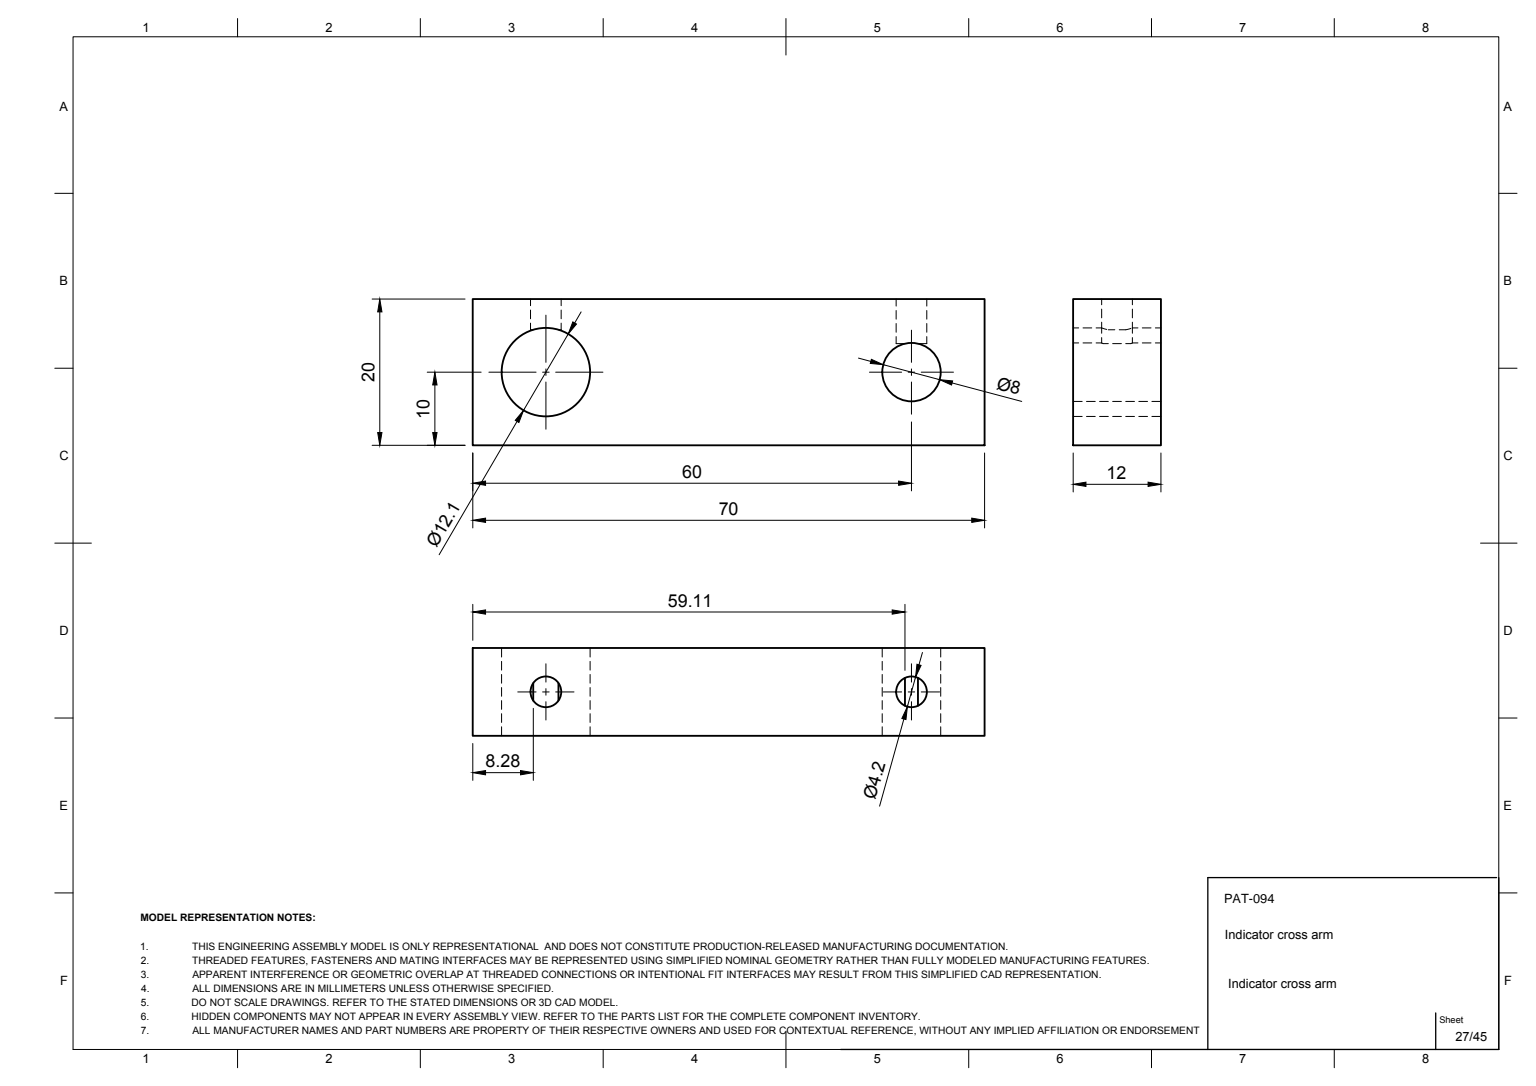
ISO-10303-21;
HEADER;
/* Generated by software containing ST-Developer
 * from STEP Tools, Inc. (www.steptools.com) 
 */

FILE_DESCRIPTION(
/* description */ ('Shaft runout checking stand'),
/* implementation_level */ '2;1');

FILE_NAME(
/* name */ 'Indicator cross arm.step',
/* time_stamp */ '2026-11-02T21:12:33-08:00',
/* author */ (''),
/* organization */ (''),
/* preprocessor_version */ 'ST-DEVELOPER v20.2',
/* originating_system */ 'Autodesk Translation Framework v15.17.0.0',
/* authorisation */ '');

FILE_SCHEMA (('AUTOMOTIVE_DESIGN { 1 0 10303 214 3 1 1 }'));
ENDSEC;

DATA;
#10=MECHANICAL_DESIGN_GEOMETRIC_PRESENTATION_REPRESENTATION('',(#488),#11748);
#329=B_SPLINE_CURVE_WITH_KNOTS('',3,(#10633,#10634,#10635,#10636,#10637,
#10638,#10639,#10640,#10641,#10642),.UNSPECIFIED.,.F.,.F.,(4,2,2,2,4),(0.882019934661292,
0.890219855506043,0.970998038219416,1.05177622093279,1.05997614177754),
 .UNSPECIFIED.);
#330=B_SPLINE_CURVE_WITH_KNOTS('',3,(#10645,#10646,#10647,#10648,#10649,
#10650,#10651,#10652,#10653,#10654),.UNSPECIFIED.,.F.,.F.,(4,2,2,2,4),(0.234687909181681,
0.242887830026432,0.323666012739805,0.404444195453179,0.41264411629793),
 .UNSPECIFIED.);
#331=B_SPLINE_CURVE_WITH_KNOTS('',3,(#10669,#10670,#10671,#10672,#10673,
#10674,#10675,#10676,#10677,#10678,#10679,#10680,#10681,#10682),
 .UNSPECIFIED.,.F.,.F.,(4,2,2,2,2,2,4),(0.761877411255191,0.798325568640294,
0.878131747417165,0.957937926194035,1.03774410497091,1.11755028374778,1.15399844113288),
 .UNSPECIFIED.);
#332=B_SPLINE_CURVE_WITH_KNOTS('',3,(#10685,#10686,#10687,#10688,#10689,
#10690,#10691,#10692,#10693,#10694,#10695,#10696,#10697,#10698),
 .UNSPECIFIED.,.F.,.F.,(4,2,2,2,2,2,4),(0.123252127125832,0.159700284510937,
0.239506463287808,0.319312642064678,0.399118820841549,0.47892499961842,
0.515373157003523),.UNSPECIFIED.);
#402=SHAPE_REPRESENTATION_RELATIONSHIP('SRR','None',#11951,#445);
#445=ADVANCED_BREP_SHAPE_REPRESENTATION('',(#536),#11727);
#488=STYLED_ITEM('',(#12169),#536);
#536=MANIFOLD_SOLID_BREP('Body1',#6234);
#641=FACE_BOUND('',#1738,.T.);
#642=FACE_BOUND('',#1740,.T.);
#643=FACE_BOUND('',#1742,.T.);
#644=FACE_BOUND('',#1743,.T.);
#645=FACE_BOUND('',#1748,.T.);
#646=FACE_BOUND('',#1749,.T.);
#647=FACE_BOUND('',#1751,.T.);
#648=FACE_BOUND('',#1752,.T.);
#815=CIRCLE('',#7153,0.21);
#816=CIRCLE('',#7154,0.21);
#817=CIRCLE('',#7156,0.21);
#818=CIRCLE('',#7157,0.21);
#819=CIRCLE('',#7160,0.21);
#820=CIRCLE('',#7161,0.21);
#821=CIRCLE('',#7163,0.21);
#822=CIRCLE('',#7164,0.21);
#823=CIRCLE('',#7167,0.4);
#824=CIRCLE('',#7168,0.4);
#825=CIRCLE('',#7170,0.605);
#826=CIRCLE('',#7171,0.605);
#1003=CYLINDRICAL_SURFACE('',#7155,0.21);
#1004=CYLINDRICAL_SURFACE('',#7162,0.21);
#1005=CYLINDRICAL_SURFACE('',#7166,0.4);
#1006=CYLINDRICAL_SURFACE('',#7169,0.605);
#1284=FACE_OUTER_BOUND('',#1731,.T.);
#1285=FACE_OUTER_BOUND('',#1732,.T.);
#1286=FACE_OUTER_BOUND('',#1733,.T.);
#1287=FACE_OUTER_BOUND('',#1734,.T.);
#1288=FACE_OUTER_BOUND('',#1735,.T.);
#1289=FACE_OUTER_BOUND('',#1736,.T.);
#1290=FACE_OUTER_BOUND('',#1737,.T.);
#1291=FACE_OUTER_BOUND('',#1739,.T.);
#1292=FACE_OUTER_BOUND('',#1741,.T.);
#1293=FACE_OUTER_BOUND('',#1744,.T.);
#1294=FACE_OUTER_BOUND('',#1745,.T.);
#1295=FACE_OUTER_BOUND('',#1746,.T.);
#1296=FACE_OUTER_BOUND('',#1747,.T.);
#1297=FACE_OUTER_BOUND('',#1750,.T.);
#1731=EDGE_LOOP('',(#5142,#5143,#5144));
#1732=EDGE_LOOP('',(#5145,#5146,#5147,#5148,#5149,#5150,#5151,#5152));
#1733=EDGE_LOOP('',(#5153,#5154));
#1734=EDGE_LOOP('',(#5155,#5156,#5157));
#1735=EDGE_LOOP('',(#5158,#5159,#5160,#5161,#5162,#5163,#5164,#5165));
#1736=EDGE_LOOP('',(#5166,#5167));
#1737=EDGE_LOOP('',(#5168,#5169,#5170,#5171));
#1738=EDGE_LOOP('',(#5172,#5173,#5174,#5175));
#1739=EDGE_LOOP('',(#5176,#5177,#5178,#5179));
#1740=EDGE_LOOP('',(#5180,#5181,#5182,#5183));
#1741=EDGE_LOOP('',(#5184,#5185,#5186,#5187));
#1742=EDGE_LOOP('',(#5188));
#1743=EDGE_LOOP('',(#5189));
#1744=EDGE_LOOP('',(#5190,#5191,#5192,#5193));
#1745=EDGE_LOOP('',(#5194,#5195,#5196,#5197));
#1746=EDGE_LOOP('',(#5198,#5199,#5200,#5201));
#1747=EDGE_LOOP('',(#5202,#5203,#5204,#5205));
#1748=EDGE_LOOP('',(#5206));
#1749=EDGE_LOOP('',(#5207));
#1750=EDGE_LOOP('',(#5208,#5209,#5210,#5211));
#1751=EDGE_LOOP('',(#5212));
#1752=EDGE_LOOP('',(#5213));
#2268=LINE('',#10627,#2735);
#2269=LINE('',#10656,#2736);
#2270=LINE('',#10659,#2737);
#2271=LINE('',#10663,#2738);
#2272=LINE('',#10700,#2739);
#2273=LINE('',#10703,#2740);
#2274=LINE('',#10708,#2741);
#2275=LINE('',#10714,#2742);
#2276=LINE('',#10719,#2743);
#2277=LINE('',#10721,#2744);
#2278=LINE('',#10723,#2745);
#2279=LINE('',#10724,#2746);
#2280=LINE('',#10727,#2747);
#2281=LINE('',#10729,#2748);
#2282=LINE('',#10730,#2749);
#2283=LINE('',#10733,#2750);
#2284=LINE('',#10735,#2751);
#2285=LINE('',#10736,#2752);
#2286=LINE('',#10738,#2753);
#2287=LINE('',#10739,#2754);
#2735=VECTOR('',#8713,1.);
#2736=VECTOR('',#8722,0.21);
#2737=VECTOR('',#8727,1.);
#2738=VECTOR('',#8730,1.);
#2739=VECTOR('',#8739,0.21);
#2740=VECTOR('',#8744,1.);
#2741=VECTOR('',#8749,0.4);
#2742=VECTOR('',#8756,0.605000000000001);
#2743=VECTOR('',#8761,1.);
#2744=VECTOR('',#8762,1.);
#2745=VECTOR('',#8763,1.);
#2746=VECTOR('',#8764,1.);
#2747=VECTOR('',#8767,1.);
#2748=VECTOR('',#8768,1.);
#2749=VECTOR('',#8769,1.);
#2750=VECTOR('',#8772,1.);
#2751=VECTOR('',#8773,1.);
#2752=VECTOR('',#8774,1.);
#2753=VECTOR('',#8777,1.);
#2754=VECTOR('',#8778,1.);
#3167=VERTEX_POINT('',#10625);
#3168=VERTEX_POINT('',#10626);
#3169=VERTEX_POINT('',#10628);
#3170=VERTEX_POINT('',#10632);
#3171=VERTEX_POINT('',#10643);
#3172=VERTEX_POINT('',#10655);
#3173=VERTEX_POINT('',#10661);
#3174=VERTEX_POINT('',#10662);
#3175=VERTEX_POINT('',#10664);
#3176=VERTEX_POINT('',#10668);
#3177=VERTEX_POINT('',#10683);
#3178=VERTEX_POINT('',#10699);
#3179=VERTEX_POINT('',#10705);
#3180=VERTEX_POINT('',#10707);
#3181=VERTEX_POINT('',#10711);
#3182=VERTEX_POINT('',#10713);
#3183=VERTEX_POINT('',#10717);
#3184=VERTEX_POINT('',#10718);
#3185=VERTEX_POINT('',#10720);
#3186=VERTEX_POINT('',#10722);
#3187=VERTEX_POINT('',#10726);
#3188=VERTEX_POINT('',#10728);
#3189=VERTEX_POINT('',#10732);
#3190=VERTEX_POINT('',#10734);
#3857=EDGE_CURVE('',#3167,#3168,#2268,.T.);
#3858=EDGE_CURVE('',#3167,#3169,#815,.T.);
#3859=EDGE_CURVE('',#3169,#3168,#816,.T.);
#3860=EDGE_CURVE('',#3170,#3167,#329,.T.);
#3861=EDGE_CURVE('',#3171,#3170,#817,.T.);
#3862=EDGE_CURVE('',#3168,#3171,#330,.T.);
#3863=EDGE_CURVE('',#3169,#3172,#2269,.T.);
#3864=EDGE_CURVE('',#3172,#3172,#818,.T.);
#3865=EDGE_CURVE('',#3171,#3170,#2270,.T.);
#3866=EDGE_CURVE('',#3173,#3174,#2271,.T.);
#3867=EDGE_CURVE('',#3173,#3175,#819,.T.);
#3868=EDGE_CURVE('',#3175,#3174,#820,.T.);
#3869=EDGE_CURVE('',#3176,#3173,#331,.T.);
#3870=EDGE_CURVE('',#3177,#3176,#821,.T.);
#3871=EDGE_CURVE('',#3174,#3177,#332,.T.);
#3872=EDGE_CURVE('',#3175,#3178,#2272,.T.);
#3873=EDGE_CURVE('',#3178,#3178,#822,.T.);
#3874=EDGE_CURVE('',#3177,#3176,#2273,.T.);
#3875=EDGE_CURVE('',#3179,#3179,#823,.T.);
#3876=EDGE_CURVE('',#3179,#3180,#2274,.T.);
#3877=EDGE_CURVE('',#3180,#3180,#824,.T.);
#3878=EDGE_CURVE('',#3181,#3181,#825,.T.);
#3879=EDGE_CURVE('',#3181,#3182,#2275,.T.);
#3880=EDGE_CURVE('',#3182,#3182,#826,.T.);
#3881=EDGE_CURVE('',#3183,#3184,#2276,.T.);
#3882=EDGE_CURVE('',#3184,#3185,#2277,.T.);
#3883=EDGE_CURVE('',#3186,#3185,#2278,.T.);
#3884=EDGE_CURVE('',#3183,#3186,#2279,.T.);
#3885=EDGE_CURVE('',#3187,#3183,#2280,.T.);
#3886=EDGE_CURVE('',#3188,#3186,#2281,.T.);
#3887=EDGE_CURVE('',#3187,#3188,#2282,.T.);
#3888=EDGE_CURVE('',#3189,#3187,#2283,.T.);
#3889=EDGE_CURVE('',#3190,#3188,#2284,.T.);
#3890=EDGE_CURVE('',#3189,#3190,#2285,.T.);
#3891=EDGE_CURVE('',#3184,#3189,#2286,.T.);
#3892=EDGE_CURVE('',#3185,#3190,#2287,.T.);
#5142=ORIENTED_EDGE('',*,*,#3857,.F.);
#5143=ORIENTED_EDGE('',*,*,#3858,.T.);
#5144=ORIENTED_EDGE('',*,*,#3859,.T.);
#5145=ORIENTED_EDGE('',*,*,#3860,.F.);
#5146=ORIENTED_EDGE('',*,*,#3861,.F.);
#5147=ORIENTED_EDGE('',*,*,#3862,.F.);
#5148=ORIENTED_EDGE('',*,*,#3859,.F.);
#5149=ORIENTED_EDGE('',*,*,#3863,.T.);
#5150=ORIENTED_EDGE('',*,*,#3864,.F.);
#5151=ORIENTED_EDGE('',*,*,#3863,.F.);
#5152=ORIENTED_EDGE('',*,*,#3858,.F.);
#5153=ORIENTED_EDGE('',*,*,#3865,.F.);
#5154=ORIENTED_EDGE('',*,*,#3861,.T.);
#5155=ORIENTED_EDGE('',*,*,#3866,.F.);
#5156=ORIENTED_EDGE('',*,*,#3867,.T.);
#5157=ORIENTED_EDGE('',*,*,#3868,.T.);
#5158=ORIENTED_EDGE('',*,*,#3869,.F.);
#5159=ORIENTED_EDGE('',*,*,#3870,.F.);
#5160=ORIENTED_EDGE('',*,*,#3871,.F.);
#5161=ORIENTED_EDGE('',*,*,#3868,.F.);
#5162=ORIENTED_EDGE('',*,*,#3872,.T.);
#5163=ORIENTED_EDGE('',*,*,#3873,.F.);
#5164=ORIENTED_EDGE('',*,*,#3872,.F.);
#5165=ORIENTED_EDGE('',*,*,#3867,.F.);
#5166=ORIENTED_EDGE('',*,*,#3874,.F.);
#5167=ORIENTED_EDGE('',*,*,#3870,.T.);
#5168=ORIENTED_EDGE('',*,*,#3875,.F.);
#5169=ORIENTED_EDGE('',*,*,#3876,.T.);
#5170=ORIENTED_EDGE('',*,*,#3877,.F.);
#5171=ORIENTED_EDGE('',*,*,#3876,.F.);
#5172=ORIENTED_EDGE('',*,*,#3862,.T.);
#5173=ORIENTED_EDGE('',*,*,#3865,.T.);
#5174=ORIENTED_EDGE('',*,*,#3860,.T.);
#5175=ORIENTED_EDGE('',*,*,#3857,.T.);
#5176=ORIENTED_EDGE('',*,*,#3878,.F.);
#5177=ORIENTED_EDGE('',*,*,#3879,.T.);
#5178=ORIENTED_EDGE('',*,*,#3880,.F.);
#5179=ORIENTED_EDGE('',*,*,#3879,.F.);
#5180=ORIENTED_EDGE('',*,*,#3871,.T.);
#5181=ORIENTED_EDGE('',*,*,#3874,.T.);
#5182=ORIENTED_EDGE('',*,*,#3869,.T.);
#5183=ORIENTED_EDGE('',*,*,#3866,.T.);
#5184=ORIENTED_EDGE('',*,*,#3881,.T.);
#5185=ORIENTED_EDGE('',*,*,#3882,.T.);
#5186=ORIENTED_EDGE('',*,*,#3883,.F.);
#5187=ORIENTED_EDGE('',*,*,#3884,.F.);
#5188=ORIENTED_EDGE('',*,*,#3864,.T.);
#5189=ORIENTED_EDGE('',*,*,#3873,.T.);
#5190=ORIENTED_EDGE('',*,*,#3885,.T.);
#5191=ORIENTED_EDGE('',*,*,#3884,.T.);
#5192=ORIENTED_EDGE('',*,*,#3886,.F.);
#5193=ORIENTED_EDGE('',*,*,#3887,.F.);
#5194=ORIENTED_EDGE('',*,*,#3888,.T.);
#5195=ORIENTED_EDGE('',*,*,#3887,.T.);
#5196=ORIENTED_EDGE('',*,*,#3889,.F.);
#5197=ORIENTED_EDGE('',*,*,#3890,.F.);
#5198=ORIENTED_EDGE('',*,*,#3891,.T.);
#5199=ORIENTED_EDGE('',*,*,#3890,.T.);
#5200=ORIENTED_EDGE('',*,*,#3892,.F.);
#5201=ORIENTED_EDGE('',*,*,#3882,.F.);
#5202=ORIENTED_EDGE('',*,*,#3892,.T.);
#5203=ORIENTED_EDGE('',*,*,#3889,.T.);
#5204=ORIENTED_EDGE('',*,*,#3886,.T.);
#5205=ORIENTED_EDGE('',*,*,#3883,.T.);
#5206=ORIENTED_EDGE('',*,*,#3877,.T.);
#5207=ORIENTED_EDGE('',*,*,#3880,.T.);
#5208=ORIENTED_EDGE('',*,*,#3891,.F.);
#5209=ORIENTED_EDGE('',*,*,#3881,.F.);
#5210=ORIENTED_EDGE('',*,*,#3885,.F.);
#5211=ORIENTED_EDGE('',*,*,#3888,.F.);
#5212=ORIENTED_EDGE('',*,*,#3875,.T.);
#5213=ORIENTED_EDGE('',*,*,#3878,.T.);
#5775=PLANE('',#7152);
#5776=PLANE('',#7158);
#5777=PLANE('',#7159);
#5778=PLANE('',#7165);
#5779=PLANE('',#7172);
#5780=PLANE('',#7173);
#5781=PLANE('',#7174);
#5782=PLANE('',#7175);
#5783=PLANE('',#7176);
#5784=PLANE('',#7177);
#6084=ADVANCED_FACE('',(#1284),#5775,.T.);
#6085=ADVANCED_FACE('',(#1285),#1003,.F.);
#6086=ADVANCED_FACE('',(#1286),#5776,.T.);
#6087=ADVANCED_FACE('',(#1287),#5777,.T.);
#6088=ADVANCED_FACE('',(#1288),#1004,.F.);
#6089=ADVANCED_FACE('',(#1289),#5778,.T.);
#6090=ADVANCED_FACE('',(#1290,#641),#1005,.F.);
#6091=ADVANCED_FACE('',(#1291,#642),#1006,.F.);
#6092=ADVANCED_FACE('',(#1292,#643,#644),#5779,.T.);
#6093=ADVANCED_FACE('',(#1293),#5780,.T.);
#6094=ADVANCED_FACE('',(#1294),#5781,.T.);
#6095=ADVANCED_FACE('',(#1295),#5782,.T.);
#6096=ADVANCED_FACE('',(#1296,#645,#646),#5783,.T.);
#6097=ADVANCED_FACE('',(#1297,#647,#648),#5784,.F.);
#6234=CLOSED_SHELL('',(#6084,#6085,#6086,#6087,#6088,#6089,#6090,#6091,
#6092,#6093,#6094,#6095,#6096,#6097));
#7151=AXIS2_PLACEMENT_3D('',#10623,#8709,#8710);
#7152=AXIS2_PLACEMENT_3D('',#10624,#8711,#8712);
#7153=AXIS2_PLACEMENT_3D('',#10629,#8714,#8715);
#7154=AXIS2_PLACEMENT_3D('',#10630,#8716,#8717);
#7155=AXIS2_PLACEMENT_3D('',#10631,#8718,#8719);
#7156=AXIS2_PLACEMENT_3D('',#10644,#8720,#8721);
#7157=AXIS2_PLACEMENT_3D('',#10657,#8723,#8724);
#7158=AXIS2_PLACEMENT_3D('',#10658,#8725,#8726);
#7159=AXIS2_PLACEMENT_3D('',#10660,#8728,#8729);
#7160=AXIS2_PLACEMENT_3D('',#10665,#8731,#8732);
#7161=AXIS2_PLACEMENT_3D('',#10666,#8733,#8734);
#7162=AXIS2_PLACEMENT_3D('',#10667,#8735,#8736);
#7163=AXIS2_PLACEMENT_3D('',#10684,#8737,#8738);
#7164=AXIS2_PLACEMENT_3D('',#10701,#8740,#8741);
#7165=AXIS2_PLACEMENT_3D('',#10702,#8742,#8743);
#7166=AXIS2_PLACEMENT_3D('',#10704,#8745,#8746);
#7167=AXIS2_PLACEMENT_3D('',#10706,#8747,#8748);
#7168=AXIS2_PLACEMENT_3D('',#10709,#8750,#8751);
#7169=AXIS2_PLACEMENT_3D('',#10710,#8752,#8753);
#7170=AXIS2_PLACEMENT_3D('',#10712,#8754,#8755);
#7171=AXIS2_PLACEMENT_3D('',#10715,#8757,#8758);
#7172=AXIS2_PLACEMENT_3D('',#10716,#8759,#8760);
#7173=AXIS2_PLACEMENT_3D('',#10725,#8765,#8766);
#7174=AXIS2_PLACEMENT_3D('',#10731,#8770,#8771);
#7175=AXIS2_PLACEMENT_3D('',#10737,#8775,#8776);
#7176=AXIS2_PLACEMENT_3D('',#10740,#8779,#8780);
#7177=AXIS2_PLACEMENT_3D('',#10741,#8781,#8782);
#8709=DIRECTION('axis',(0.,0.,1.));
#8710=DIRECTION('refdir',(1.,0.,0.));
#8711=DIRECTION('center_axis',(0.,1.,0.));
#8712=DIRECTION('ref_axis',(1.,0.,0.));
#8713=DIRECTION('',(0.,0.,1.));
#8714=DIRECTION('center_axis',(0.,1.,0.));
#8715=DIRECTION('ref_axis',(1.,0.,0.));
#8716=DIRECTION('center_axis',(0.,1.,0.));
#8717=DIRECTION('ref_axis',(1.,0.,0.));
#8718=DIRECTION('center_axis',(0.,1.,0.));
#8719=DIRECTION('ref_axis',(1.,0.,0.));
#8720=DIRECTION('center_axis',(0.,1.,0.));
#8721=DIRECTION('ref_axis',(1.,0.,0.));
#8722=DIRECTION('',(0.,1.,0.));
#8723=DIRECTION('center_axis',(0.,-1.,0.));
#8724=DIRECTION('ref_axis',(1.,0.,0.));
#8725=DIRECTION('center_axis',(0.,1.,0.));
#8726=DIRECTION('ref_axis',(1.,0.,0.));
#8727=DIRECTION('',(0.,0.,-1.));
#8728=DIRECTION('center_axis',(0.,1.,0.));
#8729=DIRECTION('ref_axis',(1.,0.,0.));
#8730=DIRECTION('',(0.,0.,1.));
#8731=DIRECTION('center_axis',(0.,1.,0.));
#8732=DIRECTION('ref_axis',(1.,0.,0.));
#8733=DIRECTION('center_axis',(0.,1.,0.));
#8734=DIRECTION('ref_axis',(1.,0.,0.));
#8735=DIRECTION('center_axis',(0.,1.,0.));
#8736=DIRECTION('ref_axis',(1.,0.,0.));
#8737=DIRECTION('center_axis',(0.,1.,0.));
#8738=DIRECTION('ref_axis',(1.,0.,0.));
#8739=DIRECTION('',(0.,1.,0.));
#8740=DIRECTION('center_axis',(0.,-1.,0.));
#8741=DIRECTION('ref_axis',(1.,0.,0.));
#8742=DIRECTION('center_axis',(0.,1.,0.));
#8743=DIRECTION('ref_axis',(1.,0.,0.));
#8744=DIRECTION('',(0.,0.,-1.));
#8745=DIRECTION('center_axis',(0.,0.,1.));
#8746=DIRECTION('ref_axis',(1.,0.,0.));
#8747=DIRECTION('center_axis',(0.,0.,1.));
#8748=DIRECTION('ref_axis',(1.,0.,0.));
#8749=DIRECTION('',(0.,0.,1.));
#8750=DIRECTION('center_axis',(0.,0.,-1.));
#8751=DIRECTION('ref_axis',(1.,0.,0.));
#8752=DIRECTION('center_axis',(0.,0.,1.));
#8753=DIRECTION('ref_axis',(1.,0.,0.));
#8754=DIRECTION('center_axis',(0.,0.,1.));
#8755=DIRECTION('ref_axis',(1.,0.,0.));
#8756=DIRECTION('',(0.,0.,1.));
#8757=DIRECTION('center_axis',(0.,0.,-1.));
#8758=DIRECTION('ref_axis',(1.,0.,0.));
#8759=DIRECTION('center_axis',(0.,1.,0.));
#8760=DIRECTION('ref_axis',(-1.,0.,0.));
#8761=DIRECTION('',(-1.,0.,0.));
#8762=DIRECTION('',(0.,0.,1.));
#8763=DIRECTION('',(-1.,0.,0.));
#8764=DIRECTION('',(0.,0.,1.));
#8765=DIRECTION('center_axis',(1.,0.,0.));
#8766=DIRECTION('ref_axis',(0.,1.,0.));
#8767=DIRECTION('',(0.,1.,0.));
#8768=DIRECTION('',(0.,1.,0.));
#8769=DIRECTION('',(0.,0.,1.));
#8770=DIRECTION('center_axis',(0.,-1.,0.));
#8771=DIRECTION('ref_axis',(1.,0.,0.));
#8772=DIRECTION('',(1.,0.,0.));
#8773=DIRECTION('',(1.,0.,0.));
#8774=DIRECTION('',(0.,0.,1.));
#8775=DIRECTION('center_axis',(-1.,0.,0.));
#8776=DIRECTION('ref_axis',(0.,-1.,0.));
#8777=DIRECTION('',(0.,-1.,0.));
#8778=DIRECTION('',(0.,-1.,0.));
#8779=DIRECTION('center_axis',(0.,0.,1.));
#8780=DIRECTION('ref_axis',(1.,0.,0.));
#8781=DIRECTION('center_axis',(0.,0.,1.));
#8782=DIRECTION('ref_axis',(1.,0.,0.));
#10623=CARTESIAN_POINT('',(0.,0.,0.));
#10624=CARTESIAN_POINT('Origin',(0.,0.39,12.6));
#10625=CARTESIAN_POINT('',(-0.088881944173156,0.39,12.4097370240956));
#10626=CARTESIAN_POINT('',(-0.088881944173156,0.39,12.7902629759044));
#10627=CARTESIAN_POINT('',(-0.088881944173156,0.39,11.9));
#10628=CARTESIAN_POINT('',(-0.21,0.39,12.6));
#10629=CARTESIAN_POINT('Origin',(0.,0.39,12.6));
#10630=CARTESIAN_POINT('Origin',(0.,0.39,12.6));
#10631=CARTESIAN_POINT('Origin',(0.,0.39,12.6));
#10632=CARTESIAN_POINT('',(0.088881944173156,0.39,12.4097370240956));
#10633=CARTESIAN_POINT('Ctrl Pts',(0.088881944173156,0.39,12.4097370240956));
#10634=CARTESIAN_POINT('Ctrl Pts',(0.086315498079388,0.390584899278025,
12.4085381007772));
#10635=CARTESIAN_POINT('Ctrl Pts',(0.0837209983713384,0.391149522707465,
12.4073893629036));
#10636=CARTESIAN_POINT('Ctrl Pts',(0.0552990416535447,0.397034429112172,
12.3954896015193));
#10637=CARTESIAN_POINT('Ctrl Pts',(0.0269260609044579,0.4,12.39));
#10638=CARTESIAN_POINT('Ctrl Pts',(-0.0269260609044578,0.4,12.39));
#10639=CARTESIAN_POINT('Ctrl Pts',(-0.0552990416535446,0.397034429112172,
12.3954896015193));
#10640=CARTESIAN_POINT('Ctrl Pts',(-0.0837209983713383,0.391149522707465,
12.4073893629036));
#10641=CARTESIAN_POINT('Ctrl Pts',(-0.086315498079388,0.390584899278025,
12.4085381007772));
#10642=CARTESIAN_POINT('Ctrl Pts',(-0.088881944173156,0.39,12.4097370240956));
#10643=CARTESIAN_POINT('',(0.088881944173156,0.39,12.7902629759044));
#10644=CARTESIAN_POINT('Origin',(0.,0.39,12.6));
#10645=CARTESIAN_POINT('Ctrl Pts',(-0.088881944173156,0.39,12.7902629759044));
#10646=CARTESIAN_POINT('Ctrl Pts',(-0.0863154980793892,0.390584899278025,
12.7914618992227));
#10647=CARTESIAN_POINT('Ctrl Pts',(-0.0837209983713384,0.391149522707465,
12.7926106370964));
#10648=CARTESIAN_POINT('Ctrl Pts',(-0.0552990416535446,0.397034429112172,
12.8045103984807));
#10649=CARTESIAN_POINT('Ctrl Pts',(-0.0269260609044578,0.4,12.81));
#10650=CARTESIAN_POINT('Ctrl Pts',(0.0269260609044579,0.4,12.81));
#10651=CARTESIAN_POINT('Ctrl Pts',(0.0552990416535447,0.397034429112172,
12.8045103984807));
#10652=CARTESIAN_POINT('Ctrl Pts',(0.0837209983713384,0.391149522707465,
12.7926106370964));
#10653=CARTESIAN_POINT('Ctrl Pts',(0.0863154980793892,0.390584899278025,
12.7914618992227));
#10654=CARTESIAN_POINT('Ctrl Pts',(0.088881944173156,0.39,12.7902629759044));
#10655=CARTESIAN_POINT('',(-0.21,1.,12.6));
#10656=CARTESIAN_POINT('',(-0.21,0.39,12.6));
#10657=CARTESIAN_POINT('Origin',(0.,1.,12.6));
#10658=CARTESIAN_POINT('Origin',(0.,0.39,12.6));
#10659=CARTESIAN_POINT('',(0.088881944173156,0.39,11.9));
#10660=CARTESIAN_POINT('Origin',(5.,0.58,12.6));
#10661=CARTESIAN_POINT('',(4.82788085521941,0.58,12.4796879058448));
#10662=CARTESIAN_POINT('',(4.82788085521941,0.58,12.7203120941552));
#10663=CARTESIAN_POINT('',(4.82788085521941,0.58,11.9));
#10664=CARTESIAN_POINT('',(4.79,0.58,12.6));
#10665=CARTESIAN_POINT('Origin',(5.,0.58,12.6));
#10666=CARTESIAN_POINT('Origin',(5.,0.58,12.6));
#10667=CARTESIAN_POINT('Origin',(5.,0.58,12.6));
#10668=CARTESIAN_POINT('',(5.17211914478059,0.58,12.4796879058448));
#10669=CARTESIAN_POINT('Ctrl Pts',(5.17211914478059,0.58,12.4796879058448));
#10670=CARTESIAN_POINT('Ctrl Pts',(5.16494300386906,0.582129571097444,12.4694216791185));
#10671=CARTESIAN_POINT('Ctrl Pts',(5.15694888384172,0.584352756238741,12.4599640357434));
#10672=CARTESIAN_POINT('Ctrl Pts',(5.12997632363586,0.591181849259721,12.4329914755375));
#10673=CARTESIAN_POINT('Ctrl Pts',(5.10650870388547,0.596121344050056,12.4168630281897));
#10674=CARTESIAN_POINT('Ctrl Pts',(5.05482987213252,0.603074162899704,12.3953614389456));
#10675=CARTESIAN_POINT('Ctrl Pts',(5.02660205959229,0.605,12.39));
#10676=CARTESIAN_POINT('Ctrl Pts',(4.97339794040771,0.605,12.39));
#10677=CARTESIAN_POINT('Ctrl Pts',(4.94517012786748,0.603074162899704,12.3953614389456));
#10678=CARTESIAN_POINT('Ctrl Pts',(4.89349129611453,0.596121344050056,12.4168630281897));
#10679=CARTESIAN_POINT('Ctrl Pts',(4.87002367636414,0.591181849259721,12.4329914755375));
#10680=CARTESIAN_POINT('Ctrl Pts',(4.84305111615828,0.584352756238741,12.4599640357434));
#10681=CARTESIAN_POINT('Ctrl Pts',(4.83505699613094,0.582129571097444,12.4694216791185));
#10682=CARTESIAN_POINT('Ctrl Pts',(4.82788085521941,0.58,12.4796879058448));
#10683=CARTESIAN_POINT('',(5.17211914478059,0.58,12.7203120941552));
#10684=CARTESIAN_POINT('Origin',(5.,0.58,12.6));
#10685=CARTESIAN_POINT('Ctrl Pts',(4.82788085521941,0.58,12.7203120941552));
#10686=CARTESIAN_POINT('Ctrl Pts',(4.83505699613094,0.582129571097444,12.7305783208815));
#10687=CARTESIAN_POINT('Ctrl Pts',(4.84305111615828,0.584352756238741,12.7400359642566));
#10688=CARTESIAN_POINT('Ctrl Pts',(4.87002367636414,0.591181849259721,12.7670085244625));
#10689=CARTESIAN_POINT('Ctrl Pts',(4.89349129611453,0.596121344050056,12.7831369718103));
#10690=CARTESIAN_POINT('Ctrl Pts',(4.94517012786748,0.603074162899704,12.8046385610544));
#10691=CARTESIAN_POINT('Ctrl Pts',(4.97339794040771,0.605,12.81));
#10692=CARTESIAN_POINT('Ctrl Pts',(5.02660205959229,0.605,12.81));
#10693=CARTESIAN_POINT('Ctrl Pts',(5.05482987213252,0.603074162899704,12.8046385610544));
#10694=CARTESIAN_POINT('Ctrl Pts',(5.10650870388547,0.596121344050056,12.7831369718103));
#10695=CARTESIAN_POINT('Ctrl Pts',(5.12997632363586,0.591181849259721,12.7670085244625));
#10696=CARTESIAN_POINT('Ctrl Pts',(5.15694888384172,0.584352756238741,12.7400359642566));
#10697=CARTESIAN_POINT('Ctrl Pts',(5.16494300386906,0.582129571097444,12.7305783208815));
#10698=CARTESIAN_POINT('Ctrl Pts',(5.17211914478059,0.58,12.7203120941552));
#10699=CARTESIAN_POINT('',(4.79,1.,12.6));
#10700=CARTESIAN_POINT('',(4.79,0.58,12.6));
#10701=CARTESIAN_POINT('Origin',(5.,1.,12.6));
#10702=CARTESIAN_POINT('Origin',(5.,0.58,12.6));
#10703=CARTESIAN_POINT('',(5.17211914478059,0.58,11.9));
#10704=CARTESIAN_POINT('Origin',(0.,0.,11.9));
#10705=CARTESIAN_POINT('',(-0.4,-4.89858719658941E-17,12.));
#10706=CARTESIAN_POINT('Origin',(0.,0.,12.));
#10707=CARTESIAN_POINT('',(-0.4,4.89858719658941E-17,13.2));
#10708=CARTESIAN_POINT('',(-0.4,-4.89858719658941E-17,11.9));
#10709=CARTESIAN_POINT('Origin',(0.,0.,13.2));
#10710=CARTESIAN_POINT('Origin',(5.,0.,11.9));
#10711=CARTESIAN_POINT('',(4.395,-7.40911313484149E-17,12.));
#10712=CARTESIAN_POINT('Origin',(5.,0.,12.));
#10713=CARTESIAN_POINT('',(4.395,7.40911313484149E-17,13.2));
#10714=CARTESIAN_POINT('',(4.395,-7.40911313484149E-17,11.9));
#10715=CARTESIAN_POINT('Origin',(5.,0.,13.2));
#10716=CARTESIAN_POINT('Origin',(6.,1.,12.));
#10717=CARTESIAN_POINT('',(6.,1.,12.));
#10718=CARTESIAN_POINT('',(-1.,1.,12.));
#10719=CARTESIAN_POINT('',(6.,1.,12.));
#10720=CARTESIAN_POINT('',(-1.,1.,13.2));
#10721=CARTESIAN_POINT('',(-1.,1.,12.));
#10722=CARTESIAN_POINT('',(6.,1.,13.2));
#10723=CARTESIAN_POINT('',(6.,1.,13.2));
#10724=CARTESIAN_POINT('',(6.,1.,12.));
#10725=CARTESIAN_POINT('Origin',(6.,-1.,12.));
#10726=CARTESIAN_POINT('',(6.,-1.,12.));
#10727=CARTESIAN_POINT('',(6.,-1.,12.));
#10728=CARTESIAN_POINT('',(6.,-1.,13.2));
#10729=CARTESIAN_POINT('',(6.,-1.,13.2));
#10730=CARTESIAN_POINT('',(6.,-1.,12.));
#10731=CARTESIAN_POINT('Origin',(-1.,-1.,12.));
#10732=CARTESIAN_POINT('',(-1.,-1.,12.));
#10733=CARTESIAN_POINT('',(-1.,-1.,12.));
#10734=CARTESIAN_POINT('',(-1.,-1.,13.2));
#10735=CARTESIAN_POINT('',(-1.,-1.,13.2));
#10736=CARTESIAN_POINT('',(-1.,-1.,12.));
#10737=CARTESIAN_POINT('Origin',(-1.,1.,12.));
#10738=CARTESIAN_POINT('',(-1.,1.,12.));
#10739=CARTESIAN_POINT('',(-1.,1.,13.2));
#10740=CARTESIAN_POINT('Origin',(2.5,0.,13.2));
#10741=CARTESIAN_POINT('Origin',(2.5,0.,12.));
#11678=UNCERTAINTY_MEASURE_WITH_UNIT(LENGTH_MEASURE(0.001),#11749,
'DISTANCE_ACCURACY_VALUE',
'Maximum model space distance between geometric entities at asserted c
onnectivities');
#11699=UNCERTAINTY_MEASURE_WITH_UNIT(LENGTH_MEASURE(0.001),#11749,
'DISTANCE_ACCURACY_VALUE',
'Maximum model space distance between geometric entities at asserted c
onnectivities');
#11727=(
GEOMETRIC_REPRESENTATION_CONTEXT(3)
GLOBAL_UNCERTAINTY_ASSIGNED_CONTEXT((#11678))
GLOBAL_UNIT_ASSIGNED_CONTEXT((#11749,#11751,#11752))
REPRESENTATION_CONTEXT('','3D')
);
#11748=(
GEOMETRIC_REPRESENTATION_CONTEXT(3)
GLOBAL_UNCERTAINTY_ASSIGNED_CONTEXT((#11699))
GLOBAL_UNIT_ASSIGNED_CONTEXT((#11749,#11751,#11752))
REPRESENTATION_CONTEXT('','3D')
);
#11749=(
LENGTH_UNIT()
NAMED_UNIT(*)
SI_UNIT(.CENTI.,.METRE.)
);
#11751=(
NAMED_UNIT(*)
PLANE_ANGLE_UNIT()
SI_UNIT($,.RADIAN.)
);
#11752=(
NAMED_UNIT(*)
SI_UNIT($,.STERADIAN.)
SOLID_ANGLE_UNIT()
);
#11780=SHAPE_DEFINITION_REPRESENTATION(#11828,#11951);
#11828=PRODUCT_DEFINITION_SHAPE('',$,#12000);
#11951=SHAPE_REPRESENTATION('',(#7151),#11727);
#11972=PRODUCT_DEFINITION_CONTEXT('part definition',#12118,'design');
#12000=PRODUCT_DEFINITION('Indicator cross arm','Indicator cross arm',#12048,
#11972);
#12048=PRODUCT_DEFINITION_FORMATION('',$,#12147);
#12118=APPLICATION_CONTEXT(
'Core Data for Automotive Mechanical Design Process');
#12119=PRODUCT_CONTEXT('part definition',#12118,'mechanical');
#12147=PRODUCT('Indicator cross arm','Indicator cross arm',
'Indicator cross arm',(#12119));
#12169=PRESENTATION_STYLE_ASSIGNMENT((#12174));
#12174=SURFACE_STYLE_USAGE(.BOTH.,#12179);
#12179=SURFACE_SIDE_STYLE('',(#12184));
#12184=SURFACE_STYLE_FILL_AREA(#12189);
#12189=FILL_AREA_STYLE('CAD Library Painted - Engineering blue',(#12194));
#12194=FILL_AREA_STYLE_COLOUR('CAD Library Painted - Engineering blue',
#12199);
#12199=COLOUR_RGB('CAD Library Painted - Engineering blue',0.12156862745098,
0.356862745098039,0.6);
ENDSEC;
END-ISO-10303-21;
